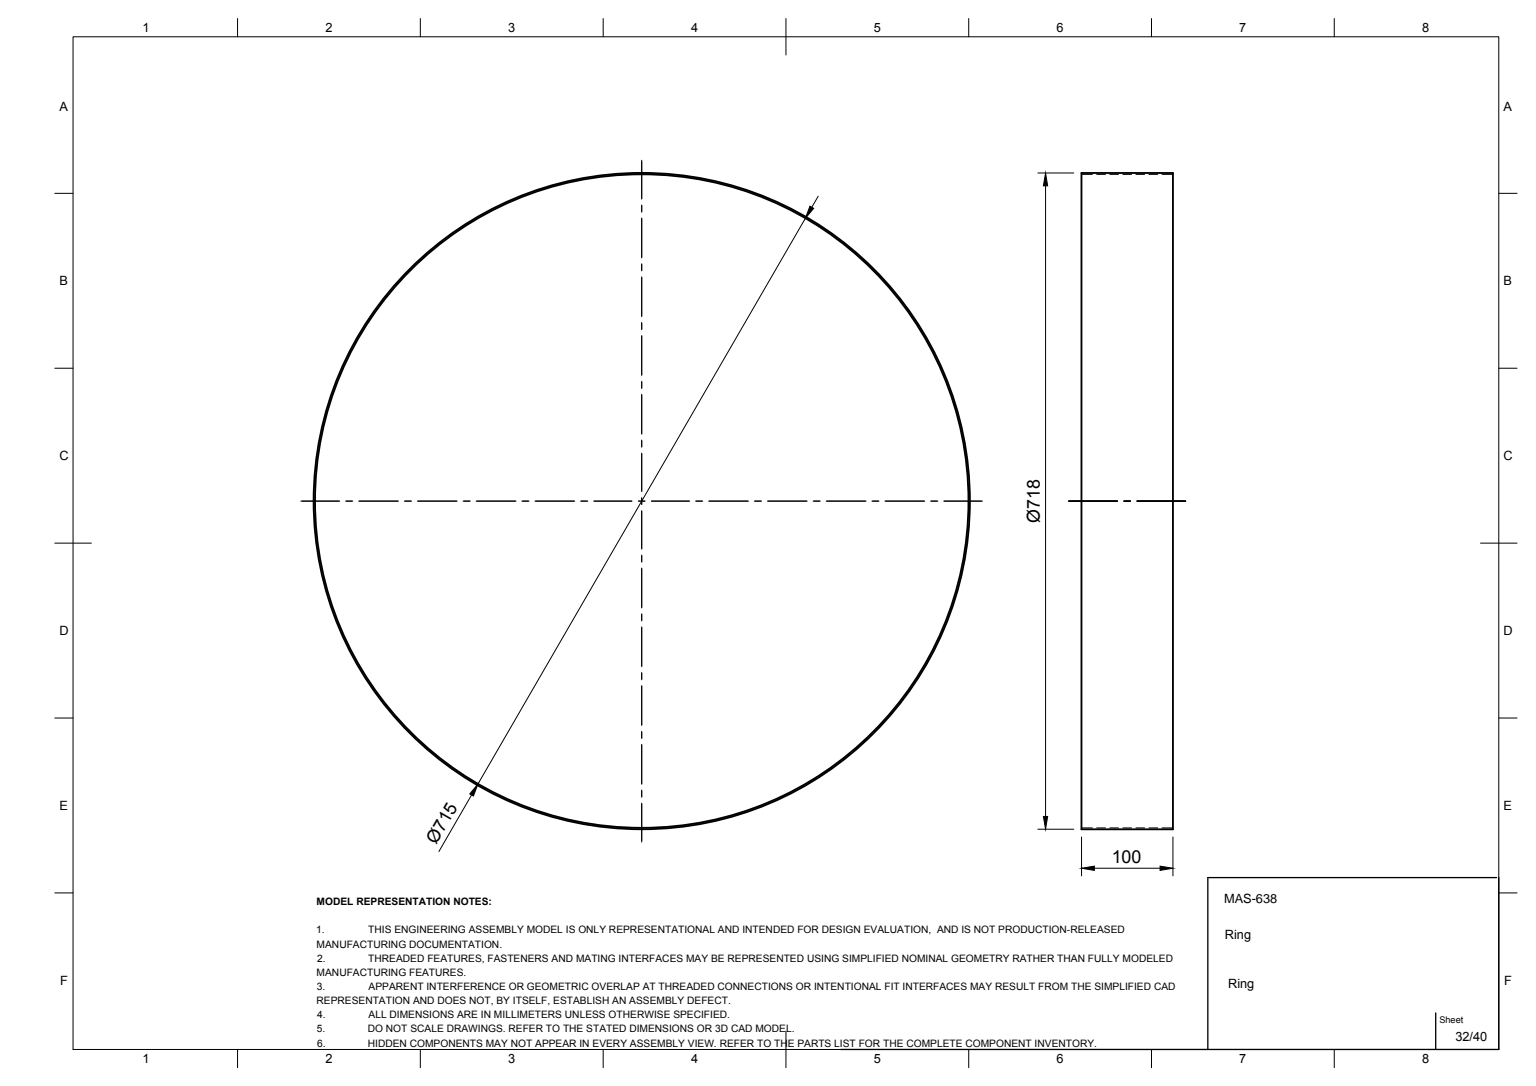
ISO-10303-21;
HEADER;
FILE_DESCRIPTION((''),'2;1');
FILE_NAME('Ring.step','2026-10-09T12:00:21-07:00',(''),(''),'','','');
FILE_SCHEMA (('AUTOMOTIVE_DESIGN { 1 0 10303 214 3 1 1 }'));
ENDSEC;
DATA;
#10=MECHANICAL_DESIGN_GEOMETRIC_PRESENTATION_REPRESENTATION('',(#429),#10334);
#145=CYLINDRICAL_SURFACE('',#4139,35.75) ;
#146=CYLINDRICAL_SURFACE('',#4142,35.9) ;
#357=SHAPE_REPRESENTATION_RELATIONSHIP('SRR','None',#10474,#389) ;
#389=ADVANCED_BREP_SHAPE_REPRESENTATION('',(#461),#10326) ;
#429=STYLED_ITEM('',(#10631),#461) ;
#461=MANIFOLD_SOLID_BREP('Body1',#3583) ;
#473=FACE_BOUND('',#1136,.T.) ;
#474=FACE_BOUND('',#1138,.T.) ;
#490=PLANE('',#4145) ;
#491=PLANE('',#4146) ;
#567=LINE('',#9663,#725) ;
#568=LINE('',#9669,#726) ;
#725=VECTOR('',#4875,35.75) ;
#726=VECTOR('',#4882,35.9) ;
#929=FACE_OUTER_BOUND('',#1133,.T.) ;
#930=FACE_OUTER_BOUND('',#1134,.T.) ;
#931=FACE_OUTER_BOUND('',#1135,.T.) ;
#932=FACE_OUTER_BOUND('',#1137,.T.) ;
#1133=EDGE_LOOP('',(#2723,#2724,#2725,#2726)) ;
#1134=EDGE_LOOP('',(#2727,#2728,#2729,#2730)) ;
#1135=EDGE_LOOP('',(#2731)) ;
#1136=EDGE_LOOP('',(#2732)) ;
#1137=EDGE_LOOP('',(#2733)) ;
#1138=EDGE_LOOP('',(#2734)) ;
#1333=CIRCLE('',#4140,35.75) ;
#1334=CIRCLE('',#4141,35.75) ;
#1335=CIRCLE('',#4143,35.9) ;
#1336=CIRCLE('',#4144,35.9) ;
#1636=VERTEX_POINT('',#9660) ;
#1637=VERTEX_POINT('',#9662) ;
#1638=VERTEX_POINT('',#9666) ;
#1639=VERTEX_POINT('',#9668) ;
#2018=EDGE_CURVE('',#1636,#1636,#1333,.T.) ;
#2019=EDGE_CURVE('',#1636,#1637,#567,.T.) ;
#2020=EDGE_CURVE('',#1637,#1637,#1334,.T.) ;
#2021=EDGE_CURVE('',#1638,#1638,#1335,.T.) ;
#2022=EDGE_CURVE('',#1638,#1639,#568,.T.) ;
#2023=EDGE_CURVE('',#1639,#1639,#1336,.T.) ;
#2723=ORIENTED_EDGE('',*,*,#2018,.T.) ;
#2724=ORIENTED_EDGE('',*,*,#2019,.T.) ;
#2725=ORIENTED_EDGE('',*,*,#2020,.F.) ;
#2726=ORIENTED_EDGE('',*,*,#2019,.F.) ;
#2727=ORIENTED_EDGE('',*,*,#2021,.T.) ;
#2728=ORIENTED_EDGE('',*,*,#2022,.T.) ;
#2729=ORIENTED_EDGE('',*,*,#2023,.F.) ;
#2730=ORIENTED_EDGE('',*,*,#2022,.F.) ;
#2731=ORIENTED_EDGE('',*,*,#2023,.T.) ;
#2732=ORIENTED_EDGE('',*,*,#2018,.F.) ;
#2733=ORIENTED_EDGE('',*,*,#2021,.F.) ;
#2734=ORIENTED_EDGE('',*,*,#2020,.T.) ;
#3437=ADVANCED_FACE('',(#929),#145,.F.) ;
#3438=ADVANCED_FACE('',(#930),#146,.T.) ;
#3439=ADVANCED_FACE('',(#931,#473),#490,.T.) ;
#3440=ADVANCED_FACE('',(#932,#474),#491,.F.) ;
#3583=CLOSED_SHELL('',(#3437,#3438,#3439,#3440)) ;
#4138=AXIS2_PLACEMENT_3D('',#9658,#4869,#4870) ;
#4139=AXIS2_PLACEMENT_3D('',#9659,#4871,#4872) ;
#4140=AXIS2_PLACEMENT_3D('',#9661,#4873,#4874) ;
#4141=AXIS2_PLACEMENT_3D('',#9664,#4876,#4877) ;
#4142=AXIS2_PLACEMENT_3D('',#9665,#4878,#4879) ;
#4143=AXIS2_PLACEMENT_3D('',#9667,#4880,#4881) ;
#4144=AXIS2_PLACEMENT_3D('',#9670,#4883,#4884) ;
#4145=AXIS2_PLACEMENT_3D('',#9671,#4885,#4886) ;
#4146=AXIS2_PLACEMENT_3D('',#9672,#4887,#4888) ;
#4869=DIRECTION('axis',(0.,0.,1.)) ;
#4870=DIRECTION('refdir',(1.,0.,0.)) ;
#4871=DIRECTION('center_axis',(7.81669040162321E-17,1.,1.01883556321148E-16)) ;
#4872=DIRECTION('ref_axis',(-1.,7.81669040162321E-17,-7.85614357465057E-33)) ;
#4873=DIRECTION('center_axis',(-7.81669040162321E-17,-1.,-1.01883556321148E-16)) ;
#4874=DIRECTION('ref_axis',(1.,-7.81669040162321E-17,7.85614357465057E-33)) ;
#4875=DIRECTION('',(7.81669040162321E-17,1.,1.01883556321148E-16)) ;
#4876=DIRECTION('center_axis',(-7.81669040162321E-17,-1.,-1.01883556321148E-16)) ;
#4877=DIRECTION('ref_axis',(1.,-7.81669040162321E-17,-7.96392216778758E-33)) ;
#4878=DIRECTION('center_axis',(7.81669040162321E-17,1.,1.01883556321148E-16)) ;
#4879=DIRECTION('ref_axis',(-1.,7.81669040162321E-17,-7.79004302140918E-33)) ;
#4880=DIRECTION('center_axis',(-7.81669040162321E-17,-1.,-1.01883556321148E-16)) ;
#4881=DIRECTION('ref_axis',(1.,-7.81669040162321E-17,-7.96392216778758E-33)) ;
#4882=DIRECTION('',(-7.81669040162321E-17,-1.,-1.01883556321148E-16)) ;
#4883=DIRECTION('center_axis',(-7.81669040162321E-17,-1.,-1.01883556321148E-16)) ;
#4884=DIRECTION('ref_axis',(1.,-7.81669040162321E-17,7.79004302140918E-33)) ;
#4885=DIRECTION('center_axis',(-7.81669040162321E-17,-1.,-1.01883556321148E-16)) ;
#4886=DIRECTION('ref_axis',(1.,-7.81669040162321E-17,1.11022302462516E-16)) ;
#4887=DIRECTION('center_axis',(-7.81669040162321E-17,-1.,-1.01883556321148E-16)) ;
#4888=DIRECTION('ref_axis',(1.,-7.81669040162321E-17,1.11022302462516E-16)) ;
#9658=CARTESIAN_POINT('',(0.,0.,0.)) ;
#9659=CARTESIAN_POINT('Origin',(23.47768801576,48.8830586252741,68.2224337400009)) ;
#9660=CARTESIAN_POINT('',(59.22768801576,48.8830586252741,68.2224337400009)) ;
#9661=CARTESIAN_POINT('Origin',(23.47768801576,48.8830586252741,68.2224337400009)) ;
#9662=CARTESIAN_POINT('',(59.22768801576,58.8830586252741,68.2224337400009)) ;
#9663=CARTESIAN_POINT('',(59.22768801576,48.8830586252741,68.2224337400009)) ;
#9664=CARTESIAN_POINT('Origin',(23.47768801576,58.8830586252741,68.2224337400009)) ;
#9665=CARTESIAN_POINT('Origin',(23.47768801576,48.8830586252741,68.2224337400009)) ;
#9666=CARTESIAN_POINT('',(59.37768801576,58.8830586252741,68.2224337400009)) ;
#9667=CARTESIAN_POINT('Origin',(23.47768801576,58.8830586252741,68.2224337400009)) ;
#9668=CARTESIAN_POINT('',(59.37768801576,48.8830586252741,68.2224337400009)) ;
#9669=CARTESIAN_POINT('',(59.37768801576,48.8830586252741,68.2224337400009)) ;
#9670=CARTESIAN_POINT('Origin',(23.47768801576,48.8830586252741,68.2224337400009)) ;
#9671=CARTESIAN_POINT('Origin',(23.47768801576,48.8830586252741,68.2224337400009)) ;
#9672=CARTESIAN_POINT('Origin',(23.47768801576,58.8830586252741,68.2224337400009)) ;
#10289=UNCERTAINTY_MEASURE_WITH_UNIT(LENGTH_MEASURE(0.001),#10335,
'DISTANCE_ACCURACY_VALUE',
'Maximum model space distance between geometric entities at asserted c
onnectivities') ;
#10297=UNCERTAINTY_MEASURE_WITH_UNIT(LENGTH_MEASURE(0.001),#10335,
'DISTANCE_ACCURACY_VALUE',
'Maximum model space distance between geometric entities at asserted c
onnectivities') ;
#10326=(
GEOMETRIC_REPRESENTATION_CONTEXT(3)
GLOBAL_UNCERTAINTY_ASSIGNED_CONTEXT((#10289))
GLOBAL_UNIT_ASSIGNED_CONTEXT((#10335,#10337,#10338))
REPRESENTATION_CONTEXT('','3D')
) ;
#10334=(
GEOMETRIC_REPRESENTATION_CONTEXT(3)
GLOBAL_UNCERTAINTY_ASSIGNED_CONTEXT((#10297))
GLOBAL_UNIT_ASSIGNED_CONTEXT((#10335,#10337,#10338))
REPRESENTATION_CONTEXT('','3D')
) ;
#10335=(
LENGTH_UNIT()
NAMED_UNIT(*)
SI_UNIT(.CENTI.,.METRE.)
) ;
#10337=(
NAMED_UNIT(*)
PLANE_ANGLE_UNIT()
SI_UNIT($,.RADIAN.)
) ;
#10338=(
NAMED_UNIT(*)
SI_UNIT($,.STERADIAN.)
SOLID_ANGLE_UNIT()
) ;
#10367=SHAPE_DEFINITION_REPRESENTATION(#10427,#10474) ;
#10427=PRODUCT_DEFINITION_SHAPE('',$,#10511) ;
#10474=SHAPE_REPRESENTATION('',(#4138),#10326) ;
#10482=PRODUCT_DEFINITION_CONTEXT('part definition',#10592,'design') ;
#10511=PRODUCT_DEFINITION('Ring','Ring',#10547,#10482) ;
#10547=PRODUCT_DEFINITION_FORMATION('',$,#10622) ;
#10592=APPLICATION_CONTEXT(
'Core Data for Automotive Mechanical Design Process') ;
#10593=PRODUCT_CONTEXT('part definition',#10592,'mechanical') ;
#10622=PRODUCT('Ring','Ring',$,(#10593)) ;
#10631=PRESENTATION_STYLE_ASSIGNMENT((#10635)) ;
#10635=SURFACE_STYLE_USAGE(.BOTH.,#10639) ;
#10639=SURFACE_SIDE_STYLE('',(#10643)) ;
#10643=SURFACE_STYLE_FILL_AREA(#10647) ;
#10647=FILL_AREA_STYLE('Opaque(25,25,25)',(#10651)) ;
#10651=FILL_AREA_STYLE_COLOUR('Opaque(25,25,25)',#10655) ;
#10655=COLOUR_RGB('Opaque(25,25,25)', 0.09019608, 0.27058824, 0.51372549) ;
ENDSEC;
END-ISO-10303-21;
